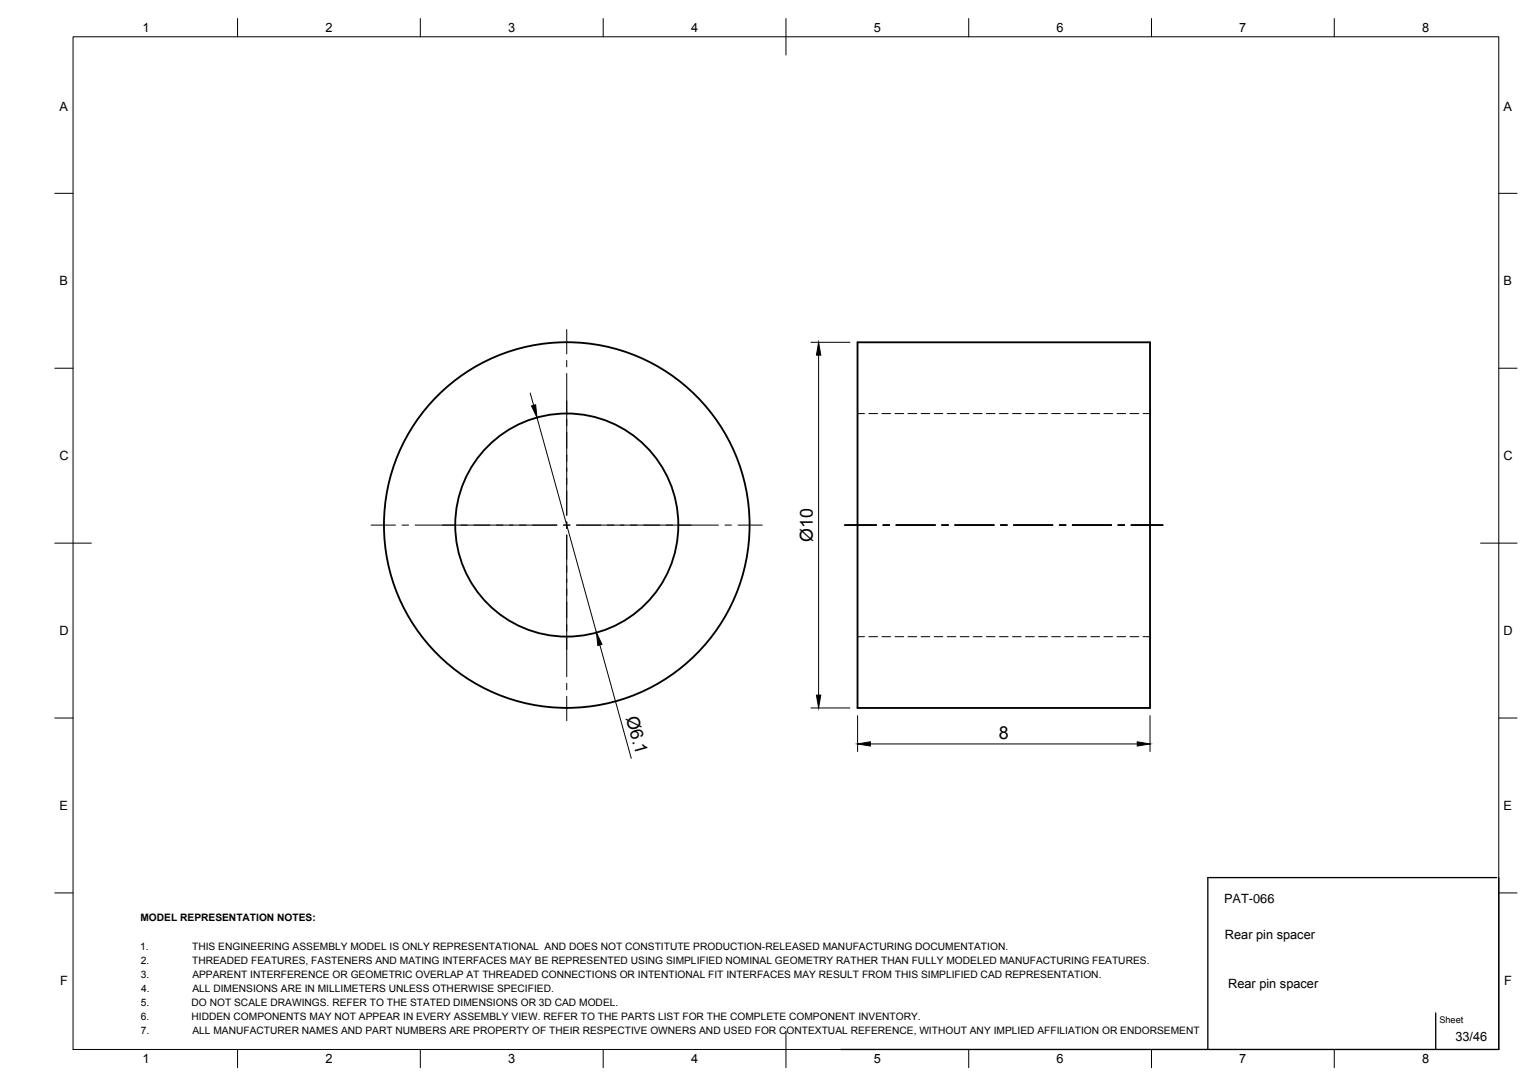
ISO-10303-21;
HEADER;
/* Generated by software containing ST-Developer
 * from STEP Tools, Inc. (www.steptools.com) 
 */

FILE_DESCRIPTION(
/* description */ ('Lever-operated bar clamp (toggle)'),
/* implementation_level */ '2;1');

FILE_NAME(
/* name */ 'Rear pin spacer.step',
/* time_stamp */ '2026-10-28T03:25:02-07:00',
/* author */ (''),
/* organization */ (''),
/* preprocessor_version */ 'ST-DEVELOPER v20.2',
/* originating_system */ 'Autodesk Translation Framework v15.17.0.0',
/* authorisation */ '');

FILE_SCHEMA (('AUTOMOTIVE_DESIGN { 1 0 10303 214 3 1 1 }'));
ENDSEC;

DATA;
#10=MECHANICAL_DESIGN_GEOMETRIC_PRESENTATION_REPRESENTATION('',(#442),#12413);
#358=SHAPE_REPRESENTATION_RELATIONSHIP('SRR','None',#12600,#396);
#396=ADVANCED_BREP_SHAPE_REPRESENTATION('',(#487),#12397);
#442=STYLED_ITEM('',(#12869),#487);
#487=MANIFOLD_SOLID_BREP('Body1',#6603);
#625=FACE_BOUND('',#1708,.T.);
#626=FACE_BOUND('',#1710,.T.);
#808=PLANE('',#7634);
#809=PLANE('',#7635);
#1174=FACE_OUTER_BOUND('',#1705,.T.);
#1175=FACE_OUTER_BOUND('',#1706,.T.);
#1176=FACE_OUTER_BOUND('',#1707,.T.);
#1177=FACE_OUTER_BOUND('',#1709,.T.);
#1705=EDGE_LOOP('',(#5575,#5576,#5577,#5578));
#1706=EDGE_LOOP('',(#5579,#5580,#5581,#5582));
#1707=EDGE_LOOP('',(#5583));
#1708=EDGE_LOOP('',(#5584));
#1709=EDGE_LOOP('',(#5585));
#1710=EDGE_LOOP('',(#5586));
#2140=LINE('',#11739,#2581);
#2141=LINE('',#11745,#2582);
#2581=VECTOR('',#9365,0.305);
#2582=VECTOR('',#9372,0.5);
#2999=CIRCLE('',#7629,0.305);
#3000=CIRCLE('',#7630,0.305);
#3001=CIRCLE('',#7632,0.5);
#3002=CIRCLE('',#7633,0.5);
#3466=VERTEX_POINT('',#11736);
#3467=VERTEX_POINT('',#11738);
#3468=VERTEX_POINT('',#11742);
#3469=VERTEX_POINT('',#11744);
#4192=EDGE_CURVE('',#3466,#3466,#2999,.T.);
#4193=EDGE_CURVE('',#3466,#3467,#2140,.T.);
#4194=EDGE_CURVE('',#3467,#3467,#3000,.T.);
#4195=EDGE_CURVE('',#3468,#3468,#3001,.T.);
#4196=EDGE_CURVE('',#3468,#3469,#2141,.T.);
#4197=EDGE_CURVE('',#3469,#3469,#3002,.T.);
#5575=ORIENTED_EDGE('',*,*,#4192,.F.);
#5576=ORIENTED_EDGE('',*,*,#4193,.T.);
#5577=ORIENTED_EDGE('',*,*,#4194,.T.);
#5578=ORIENTED_EDGE('',*,*,#4193,.F.);
#5579=ORIENTED_EDGE('',*,*,#4195,.F.);
#5580=ORIENTED_EDGE('',*,*,#4196,.T.);
#5581=ORIENTED_EDGE('',*,*,#4197,.T.);
#5582=ORIENTED_EDGE('',*,*,#4196,.F.);
#5583=ORIENTED_EDGE('',*,*,#4195,.T.);
#5584=ORIENTED_EDGE('',*,*,#4192,.T.);
#5585=ORIENTED_EDGE('',*,*,#4197,.F.);
#5586=ORIENTED_EDGE('',*,*,#4194,.F.);
#6133=CYLINDRICAL_SURFACE('',#7628,0.305);
#6134=CYLINDRICAL_SURFACE('',#7631,0.5);
#6449=ADVANCED_FACE('',(#1174),#6133,.F.);
#6450=ADVANCED_FACE('',(#1175),#6134,.T.);
#6451=ADVANCED_FACE('',(#1176,#625),#808,.T.);
#6452=ADVANCED_FACE('',(#1177,#626),#809,.F.);
#6603=CLOSED_SHELL('',(#6449,#6450,#6451,#6452));
#7627=AXIS2_PLACEMENT_3D('',#11734,#9359,#9360);
#7628=AXIS2_PLACEMENT_3D('',#11735,#9361,#9362);
#7629=AXIS2_PLACEMENT_3D('',#11737,#9363,#9364);
#7630=AXIS2_PLACEMENT_3D('',#11740,#9366,#9367);
#7631=AXIS2_PLACEMENT_3D('',#11741,#9368,#9369);
#7632=AXIS2_PLACEMENT_3D('',#11743,#9370,#9371);
#7633=AXIS2_PLACEMENT_3D('',#11746,#9373,#9374);
#7634=AXIS2_PLACEMENT_3D('',#11747,#9375,#9376);
#7635=AXIS2_PLACEMENT_3D('',#11748,#9377,#9378);
#9359=DIRECTION('axis',(0.,0.,1.));
#9360=DIRECTION('refdir',(1.,0.,0.));
#9361=DIRECTION('center_axis',(0.,1.,0.));
#9362=DIRECTION('ref_axis',(1.,0.,0.));
#9363=DIRECTION('center_axis',(0.,-1.,0.));
#9364=DIRECTION('ref_axis',(1.,0.,0.));
#9365=DIRECTION('',(0.,-1.,0.));
#9366=DIRECTION('center_axis',(0.,-1.,0.));
#9367=DIRECTION('ref_axis',(1.,0.,0.));
#9368=DIRECTION('center_axis',(0.,1.,0.));
#9369=DIRECTION('ref_axis',(1.,0.,0.));
#9370=DIRECTION('center_axis',(0.,1.,0.));
#9371=DIRECTION('ref_axis',(1.,0.,0.));
#9372=DIRECTION('',(0.,-1.,0.));
#9373=DIRECTION('center_axis',(0.,1.,0.));
#9374=DIRECTION('ref_axis',(1.,0.,0.));
#9375=DIRECTION('center_axis',(0.,1.,0.));
#9376=DIRECTION('ref_axis',(1.,0.,0.));
#9377=DIRECTION('center_axis',(0.,1.,0.));
#9378=DIRECTION('ref_axis',(1.,0.,0.));
#11734=CARTESIAN_POINT('',(0.,0.,0.));
#11735=CARTESIAN_POINT('Origin',(-2.82632109303527,-4.7,8.79263101785268));
#11736=CARTESIAN_POINT('',(-3.13132109303527,-3.9,8.79263101785268));
#11737=CARTESIAN_POINT('Origin',(-2.82632109303527,-3.9,8.79263101785268));
#11738=CARTESIAN_POINT('',(-3.13132109303527,-4.7,8.79263101785268));
#11739=CARTESIAN_POINT('',(-3.13132109303527,-4.7,8.79263101785268));
#11740=CARTESIAN_POINT('Origin',(-2.82632109303527,-4.7,8.79263101785268));
#11741=CARTESIAN_POINT('Origin',(-2.82632109303527,-4.7,8.79263101785268));
#11742=CARTESIAN_POINT('',(-3.32632109303527,-3.9,8.79263101785268));
#11743=CARTESIAN_POINT('Origin',(-2.82632109303527,-3.9,8.79263101785268));
#11744=CARTESIAN_POINT('',(-3.32632109303527,-4.7,8.79263101785268));
#11745=CARTESIAN_POINT('',(-3.32632109303527,-4.7,8.79263101785268));
#11746=CARTESIAN_POINT('Origin',(-2.82632109303527,-4.7,8.79263101785268));
#11747=CARTESIAN_POINT('Origin',(-2.82632109303527,-3.9,8.79263101785268));
#11748=CARTESIAN_POINT('Origin',(-2.82632109303527,-4.7,8.79263101785268));
#12351=UNCERTAINTY_MEASURE_WITH_UNIT(LENGTH_MEASURE(0.001),#12414,
'DISTANCE_ACCURACY_VALUE',
'Maximum model space distance between geometric entities at asserted c
onnectivities');
#12367=UNCERTAINTY_MEASURE_WITH_UNIT(LENGTH_MEASURE(0.001),#12414,
'DISTANCE_ACCURACY_VALUE',
'Maximum model space distance between geometric entities at asserted c
onnectivities');
#12397=(
GEOMETRIC_REPRESENTATION_CONTEXT(3)
GLOBAL_UNCERTAINTY_ASSIGNED_CONTEXT((#12351))
GLOBAL_UNIT_ASSIGNED_CONTEXT((#12414,#12416,#12417))
REPRESENTATION_CONTEXT('','3D')
);
#12413=(
GEOMETRIC_REPRESENTATION_CONTEXT(3)
GLOBAL_UNCERTAINTY_ASSIGNED_CONTEXT((#12367))
GLOBAL_UNIT_ASSIGNED_CONTEXT((#12414,#12416,#12417))
REPRESENTATION_CONTEXT('','3D')
);
#12414=(
LENGTH_UNIT()
NAMED_UNIT(*)
SI_UNIT(.CENTI.,.METRE.)
);
#12416=(
NAMED_UNIT(*)
PLANE_ANGLE_UNIT()
SI_UNIT($,.RADIAN.)
);
#12417=(
NAMED_UNIT(*)
SI_UNIT($,.STERADIAN.)
SOLID_ANGLE_UNIT()
);
#12447=SHAPE_DEFINITION_REPRESENTATION(#12499,#12600);
#12499=PRODUCT_DEFINITION_SHAPE('',$,#12646);
#12600=SHAPE_REPRESENTATION('',(#7627),#12397);
#12616=PRODUCT_DEFINITION_CONTEXT('part definition',#12753,'design');
#12646=PRODUCT_DEFINITION('Rear pin spacer','Rear pin spacer',#12691,#12616);
#12691=PRODUCT_DEFINITION_FORMATION('',$,#12784);
#12753=APPLICATION_CONTEXT(
'Core Data for Automotive Mechanical Design Process');
#12754=PRODUCT_CONTEXT('part definition',#12753,'mechanical');
#12784=PRODUCT('Rear pin spacer','Rear pin spacer','Rear pin spacer',(#12754));
#12863=COLOUR_RGB('Grey',0.48,0.52,0.57);
#12864=FILL_AREA_STYLE_COLOUR('',#12863);
#12865=FILL_AREA_STYLE('',(#12864));
#12866=SURFACE_STYLE_FILL_AREA(#12865);
#12867=SURFACE_SIDE_STYLE('',(#12866));
#12868=SURFACE_STYLE_USAGE(.BOTH.,#12867);
#12869=PRESENTATION_STYLE_ASSIGNMENT((#12868));
ENDSEC;
END-ISO-10303-21;
